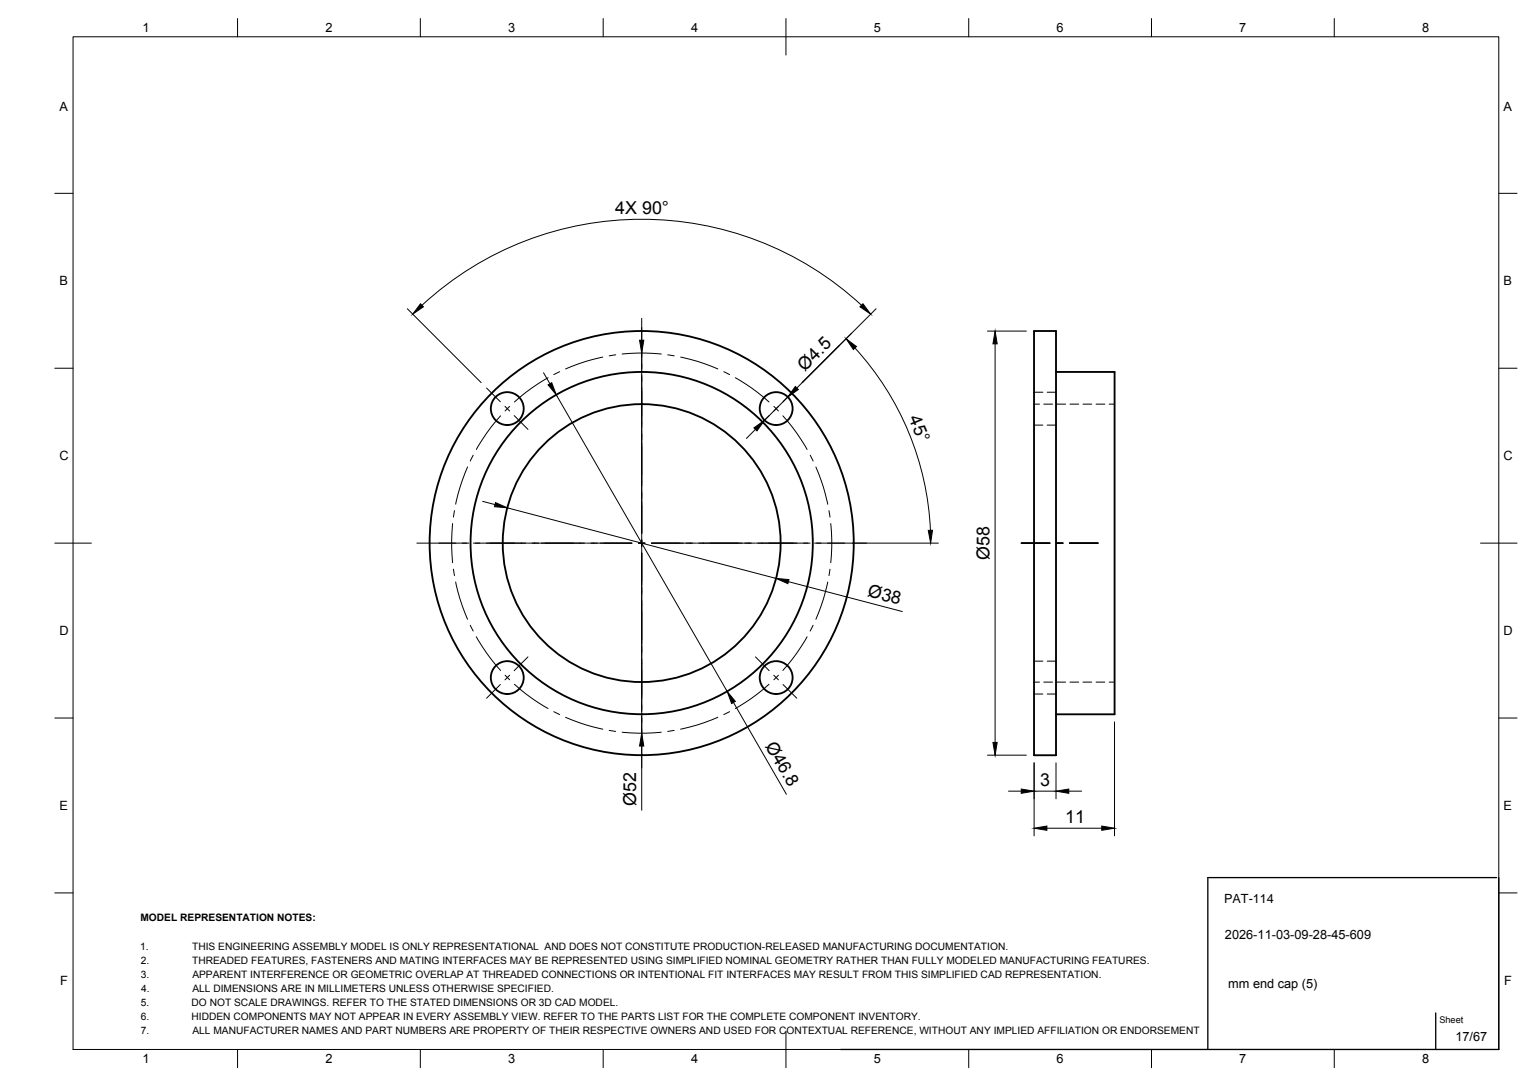
ISO-10303-21;
HEADER;
/* Generated by software containing ST-Developer
 * from STEP Tools, Inc. (www.steptools.com) 
 */

FILE_DESCRIPTION(
/* description */ ('Two-stage gear reducer in split housing'),
/* implementation_level */ '2;1');

FILE_NAME(
/* name */ 'mm end cap (5).step',
/* time_stamp */ '2026-10-28T03:22:31-07:00',
/* author */ (''),
/* organization */ (''),
/* preprocessor_version */ 'ST-DEVELOPER v20.2',
/* originating_system */ 'Autodesk Translation Framework v15.17.0.0',
/* authorisation */ '');

FILE_SCHEMA (('AUTOMOTIVE_DESIGN { 1 0 10303 214 3 1 1 }'));
ENDSEC;

DATA;
#10=MECHANICAL_DESIGN_GEOMETRIC_PRESENTATION_REPRESENTATION('',(#1246),#73366);
#1134=SHAPE_REPRESENTATION_RELATIONSHIP('SRR','None',#73621,#1190);
#1190=ADVANCED_BREP_SHAPE_REPRESENTATION('',(#1317),#73317);
#1246=STYLED_ITEM('',(#74002),#1317);
#1317=MANIFOLD_SOLID_BREP('Body1',#16134);
#1499=FACE_BOUND('',#3296,.T.);
#1500=FACE_BOUND('',#3300,.T.);
#1501=FACE_BOUND('',#3301,.T.);
#1502=FACE_BOUND('',#3302,.T.);
#1503=FACE_BOUND('',#3303,.T.);
#1504=FACE_BOUND('',#3304,.T.);
#1505=FACE_BOUND('',#3306,.T.);
#1506=FACE_BOUND('',#3307,.T.);
#1507=FACE_BOUND('',#3308,.T.);
#1508=FACE_BOUND('',#3309,.T.);
#1509=FACE_BOUND('',#3310,.T.);
#1723=PLANE('',#17350);
#1724=PLANE('',#17357);
#1725=PLANE('',#17358);
#2252=FACE_OUTER_BOUND('',#3290,.T.);
#2253=FACE_OUTER_BOUND('',#3291,.T.);
#2254=FACE_OUTER_BOUND('',#3292,.T.);
#2255=FACE_OUTER_BOUND('',#3293,.T.);
#2256=FACE_OUTER_BOUND('',#3294,.T.);
#2257=FACE_OUTER_BOUND('',#3295,.T.);
#2258=FACE_OUTER_BOUND('',#3297,.T.);
#2259=FACE_OUTER_BOUND('',#3298,.T.);
#2260=FACE_OUTER_BOUND('',#3299,.T.);
#2261=FACE_OUTER_BOUND('',#3305,.T.);
#3290=EDGE_LOOP('',(#11617,#11618,#11619,#11620));
#3291=EDGE_LOOP('',(#11621,#11622,#11623,#11624));
#3292=EDGE_LOOP('',(#11625,#11626,#11627,#11628));
#3293=EDGE_LOOP('',(#11629,#11630,#11631,#11632));
#3294=EDGE_LOOP('',(#11633,#11634,#11635,#11636));
#3295=EDGE_LOOP('',(#11637));
#3296=EDGE_LOOP('',(#11638));
#3297=EDGE_LOOP('',(#11639,#11640,#11641,#11642));
#3298=EDGE_LOOP('',(#11643,#11644,#11645,#11646));
#3299=EDGE_LOOP('',(#11647));
#3300=EDGE_LOOP('',(#11648));
#3301=EDGE_LOOP('',(#11649));
#3302=EDGE_LOOP('',(#11650));
#3303=EDGE_LOOP('',(#11651));
#3304=EDGE_LOOP('',(#11652));
#3305=EDGE_LOOP('',(#11653));
#3306=EDGE_LOOP('',(#11654));
#3307=EDGE_LOOP('',(#11655));
#3308=EDGE_LOOP('',(#11656));
#3309=EDGE_LOOP('',(#11657));
#3310=EDGE_LOOP('',(#11658));
#4353=LINE('',#23968,#5377);
#4354=LINE('',#23974,#5378);
#4355=LINE('',#23980,#5379);
#4356=LINE('',#23986,#5380);
#4357=LINE('',#23992,#5381);
#4358=LINE('',#24000,#5382);
#4359=LINE('',#24005,#5383);
#5377=VECTOR('',#19805,0.225);
#5378=VECTOR('',#19812,0.225);
#5379=VECTOR('',#19819,0.225);
#5380=VECTOR('',#19826,0.225);
#5381=VECTOR('',#19833,2.34);
#5382=VECTOR('',#19844,1.9);
#5383=VECTOR('',#19849,2.9);
#6362=CIRCLE('',#17336,0.225);
#6363=CIRCLE('',#17337,0.225);
#6364=CIRCLE('',#17339,0.225);
#6365=CIRCLE('',#17340,0.225);
#6366=CIRCLE('',#17342,0.225);
#6367=CIRCLE('',#17343,0.225);
#6368=CIRCLE('',#17345,0.225);
#6369=CIRCLE('',#17346,0.225);
#6370=CIRCLE('',#17348,2.34);
#6371=CIRCLE('',#17349,2.34);
#6372=CIRCLE('',#17351,1.9);
#6373=CIRCLE('',#17353,1.9);
#6374=CIRCLE('',#17355,2.9);
#6375=CIRCLE('',#17356,2.9);
#7194=VERTEX_POINT('',#23965);
#7195=VERTEX_POINT('',#23967);
#7196=VERTEX_POINT('',#23971);
#7197=VERTEX_POINT('',#23973);
#7198=VERTEX_POINT('',#23977);
#7199=VERTEX_POINT('',#23979);
#7200=VERTEX_POINT('',#23983);
#7201=VERTEX_POINT('',#23985);
#7202=VERTEX_POINT('',#23989);
#7203=VERTEX_POINT('',#23991);
#7204=VERTEX_POINT('',#23995);
#7205=VERTEX_POINT('',#23998);
#7206=VERTEX_POINT('',#24002);
#7207=VERTEX_POINT('',#24004);
#8862=EDGE_CURVE('',#7194,#7194,#6362,.T.);
#8863=EDGE_CURVE('',#7194,#7195,#4353,.T.);
#8864=EDGE_CURVE('',#7195,#7195,#6363,.T.);
#8865=EDGE_CURVE('',#7196,#7196,#6364,.T.);
#8866=EDGE_CURVE('',#7196,#7197,#4354,.T.);
#8867=EDGE_CURVE('',#7197,#7197,#6365,.T.);
#8868=EDGE_CURVE('',#7198,#7198,#6366,.T.);
#8869=EDGE_CURVE('',#7198,#7199,#4355,.T.);
#8870=EDGE_CURVE('',#7199,#7199,#6367,.T.);
#8871=EDGE_CURVE('',#7200,#7200,#6368,.T.);
#8872=EDGE_CURVE('',#7200,#7201,#4356,.T.);
#8873=EDGE_CURVE('',#7201,#7201,#6369,.T.);
#8874=EDGE_CURVE('',#7202,#7202,#6370,.T.);
#8875=EDGE_CURVE('',#7202,#7203,#4357,.T.);
#8876=EDGE_CURVE('',#7203,#7203,#6371,.T.);
#8877=EDGE_CURVE('',#7204,#7204,#6372,.T.);
#8878=EDGE_CURVE('',#7205,#7205,#6373,.T.);
#8879=EDGE_CURVE('',#7205,#7204,#4358,.T.);
#8880=EDGE_CURVE('',#7206,#7206,#6374,.T.);
#8881=EDGE_CURVE('',#7206,#7207,#4359,.T.);
#8882=EDGE_CURVE('',#7207,#7207,#6375,.T.);
#11617=ORIENTED_EDGE('',*,*,#8862,.F.);
#11618=ORIENTED_EDGE('',*,*,#8863,.T.);
#11619=ORIENTED_EDGE('',*,*,#8864,.F.);
#11620=ORIENTED_EDGE('',*,*,#8863,.F.);
#11621=ORIENTED_EDGE('',*,*,#8865,.F.);
#11622=ORIENTED_EDGE('',*,*,#8866,.T.);
#11623=ORIENTED_EDGE('',*,*,#8867,.F.);
#11624=ORIENTED_EDGE('',*,*,#8866,.F.);
#11625=ORIENTED_EDGE('',*,*,#8868,.F.);
#11626=ORIENTED_EDGE('',*,*,#8869,.T.);
#11627=ORIENTED_EDGE('',*,*,#8870,.F.);
#11628=ORIENTED_EDGE('',*,*,#8869,.F.);
#11629=ORIENTED_EDGE('',*,*,#8871,.F.);
#11630=ORIENTED_EDGE('',*,*,#8872,.T.);
#11631=ORIENTED_EDGE('',*,*,#8873,.F.);
#11632=ORIENTED_EDGE('',*,*,#8872,.F.);
#11633=ORIENTED_EDGE('',*,*,#8874,.F.);
#11634=ORIENTED_EDGE('',*,*,#8875,.T.);
#11635=ORIENTED_EDGE('',*,*,#8876,.T.);
#11636=ORIENTED_EDGE('',*,*,#8875,.F.);
#11637=ORIENTED_EDGE('',*,*,#8876,.F.);
#11638=ORIENTED_EDGE('',*,*,#8877,.F.);
#11639=ORIENTED_EDGE('',*,*,#8878,.F.);
#11640=ORIENTED_EDGE('',*,*,#8879,.T.);
#11641=ORIENTED_EDGE('',*,*,#8877,.T.);
#11642=ORIENTED_EDGE('',*,*,#8879,.F.);
#11643=ORIENTED_EDGE('',*,*,#8880,.F.);
#11644=ORIENTED_EDGE('',*,*,#8881,.T.);
#11645=ORIENTED_EDGE('',*,*,#8882,.T.);
#11646=ORIENTED_EDGE('',*,*,#8881,.F.);
#11647=ORIENTED_EDGE('',*,*,#8880,.T.);
#11648=ORIENTED_EDGE('',*,*,#8878,.T.);
#11649=ORIENTED_EDGE('',*,*,#8873,.T.);
#11650=ORIENTED_EDGE('',*,*,#8870,.T.);
#11651=ORIENTED_EDGE('',*,*,#8867,.T.);
#11652=ORIENTED_EDGE('',*,*,#8864,.T.);
#11653=ORIENTED_EDGE('',*,*,#8882,.F.);
#11654=ORIENTED_EDGE('',*,*,#8874,.T.);
#11655=ORIENTED_EDGE('',*,*,#8871,.T.);
#11656=ORIENTED_EDGE('',*,*,#8868,.T.);
#11657=ORIENTED_EDGE('',*,*,#8865,.T.);
#11658=ORIENTED_EDGE('',*,*,#8862,.T.);
#15036=CYLINDRICAL_SURFACE('',#17335,0.225);
#15037=CYLINDRICAL_SURFACE('',#17338,0.225);
#15038=CYLINDRICAL_SURFACE('',#17341,0.225);
#15039=CYLINDRICAL_SURFACE('',#17344,0.225);
#15040=CYLINDRICAL_SURFACE('',#17347,2.34);
#15041=CYLINDRICAL_SURFACE('',#17352,1.9);
#15042=CYLINDRICAL_SURFACE('',#17354,2.9);
#15459=ADVANCED_FACE('',(#2252),#15036,.F.);
#15460=ADVANCED_FACE('',(#2253),#15037,.F.);
#15461=ADVANCED_FACE('',(#2254),#15038,.F.);
#15462=ADVANCED_FACE('',(#2255),#15039,.F.);
#15463=ADVANCED_FACE('',(#2256),#15040,.T.);
#15464=ADVANCED_FACE('',(#2257,#1499),#1723,.F.);
#15465=ADVANCED_FACE('',(#2258),#15041,.F.);
#15466=ADVANCED_FACE('',(#2259),#15042,.T.);
#15467=ADVANCED_FACE('',(#2260,#1500,#1501,#1502,#1503,#1504),#1724,.T.);
#15468=ADVANCED_FACE('',(#2261,#1505,#1506,#1507,#1508,#1509),#1725,.F.);
#16134=CLOSED_SHELL('',(#15459,#15460,#15461,#15462,#15463,#15464,#15465,
#15466,#15467,#15468));
#17334=AXIS2_PLACEMENT_3D('',#23963,#19799,#19800);
#17335=AXIS2_PLACEMENT_3D('',#23964,#19801,#19802);
#17336=AXIS2_PLACEMENT_3D('',#23966,#19803,#19804);
#17337=AXIS2_PLACEMENT_3D('',#23969,#19806,#19807);
#17338=AXIS2_PLACEMENT_3D('',#23970,#19808,#19809);
#17339=AXIS2_PLACEMENT_3D('',#23972,#19810,#19811);
#17340=AXIS2_PLACEMENT_3D('',#23975,#19813,#19814);
#17341=AXIS2_PLACEMENT_3D('',#23976,#19815,#19816);
#17342=AXIS2_PLACEMENT_3D('',#23978,#19817,#19818);
#17343=AXIS2_PLACEMENT_3D('',#23981,#19820,#19821);
#17344=AXIS2_PLACEMENT_3D('',#23982,#19822,#19823);
#17345=AXIS2_PLACEMENT_3D('',#23984,#19824,#19825);
#17346=AXIS2_PLACEMENT_3D('',#23987,#19827,#19828);
#17347=AXIS2_PLACEMENT_3D('',#23988,#19829,#19830);
#17348=AXIS2_PLACEMENT_3D('',#23990,#19831,#19832);
#17349=AXIS2_PLACEMENT_3D('',#23993,#19834,#19835);
#17350=AXIS2_PLACEMENT_3D('',#23994,#19836,#19837);
#17351=AXIS2_PLACEMENT_3D('',#23996,#19838,#19839);
#17352=AXIS2_PLACEMENT_3D('',#23997,#19840,#19841);
#17353=AXIS2_PLACEMENT_3D('',#23999,#19842,#19843);
#17354=AXIS2_PLACEMENT_3D('',#24001,#19845,#19846);
#17355=AXIS2_PLACEMENT_3D('',#24003,#19847,#19848);
#17356=AXIS2_PLACEMENT_3D('',#24006,#19850,#19851);
#17357=AXIS2_PLACEMENT_3D('',#24007,#19852,#19853);
#17358=AXIS2_PLACEMENT_3D('',#24008,#19854,#19855);
#19799=DIRECTION('axis',(0.,0.,1.));
#19800=DIRECTION('refdir',(1.,0.,0.));
#19801=DIRECTION('center_axis',(0.,1.,0.));
#19802=DIRECTION('ref_axis',(1.,0.,0.));
#19803=DIRECTION('center_axis',(0.,1.,0.));
#19804=DIRECTION('ref_axis',(1.,0.,0.));
#19805=DIRECTION('',(0.,1.,0.));
#19806=DIRECTION('center_axis',(0.,-1.,0.));
#19807=DIRECTION('ref_axis',(1.,0.,0.));
#19808=DIRECTION('center_axis',(0.,1.,0.));
#19809=DIRECTION('ref_axis',(1.,0.,0.));
#19810=DIRECTION('center_axis',(0.,1.,0.));
#19811=DIRECTION('ref_axis',(1.,0.,0.));
#19812=DIRECTION('',(0.,1.,0.));
#19813=DIRECTION('center_axis',(0.,-1.,0.));
#19814=DIRECTION('ref_axis',(1.,0.,0.));
#19815=DIRECTION('center_axis',(0.,1.,0.));
#19816=DIRECTION('ref_axis',(1.,0.,0.));
#19817=DIRECTION('center_axis',(0.,1.,0.));
#19818=DIRECTION('ref_axis',(1.,0.,0.));
#19819=DIRECTION('',(0.,1.,0.));
#19820=DIRECTION('center_axis',(0.,-1.,0.));
#19821=DIRECTION('ref_axis',(1.,0.,0.));
#19822=DIRECTION('center_axis',(0.,1.,0.));
#19823=DIRECTION('ref_axis',(1.,0.,0.));
#19824=DIRECTION('center_axis',(0.,1.,0.));
#19825=DIRECTION('ref_axis',(1.,0.,0.));
#19826=DIRECTION('',(0.,1.,0.));
#19827=DIRECTION('center_axis',(0.,-1.,0.));
#19828=DIRECTION('ref_axis',(1.,0.,0.));
#19829=DIRECTION('center_axis',(0.,1.,0.));
#19830=DIRECTION('ref_axis',(1.,0.,0.));
#19831=DIRECTION('center_axis',(0.,1.,0.));
#19832=DIRECTION('ref_axis',(1.,0.,0.));
#19833=DIRECTION('',(0.,-1.,0.));
#19834=DIRECTION('center_axis',(0.,1.,0.));
#19835=DIRECTION('ref_axis',(1.,0.,0.));
#19836=DIRECTION('center_axis',(0.,1.,0.));
#19837=DIRECTION('ref_axis',(1.,0.,0.));
#19838=DIRECTION('center_axis',(0.,-1.,0.));
#19839=DIRECTION('ref_axis',(1.,0.,0.));
#19840=DIRECTION('center_axis',(0.,1.,0.));
#19841=DIRECTION('ref_axis',(1.,0.,0.));
#19842=DIRECTION('center_axis',(0.,-1.,0.));
#19843=DIRECTION('ref_axis',(1.,0.,0.));
#19844=DIRECTION('',(0.,-1.,0.));
#19845=DIRECTION('center_axis',(0.,1.,0.));
#19846=DIRECTION('ref_axis',(1.,0.,0.));
#19847=DIRECTION('center_axis',(0.,1.,0.));
#19848=DIRECTION('ref_axis',(1.,0.,0.));
#19849=DIRECTION('',(0.,-1.,0.));
#19850=DIRECTION('center_axis',(0.,1.,0.));
#19851=DIRECTION('ref_axis',(1.,0.,0.));
#19852=DIRECTION('center_axis',(0.,1.,0.));
#19853=DIRECTION('ref_axis',(1.,0.,0.));
#19854=DIRECTION('center_axis',(0.,1.,0.));
#19855=DIRECTION('ref_axis',(1.,0.,0.));
#23963=CARTESIAN_POINT('',(0.,0.,0.));
#23964=CARTESIAN_POINT('Origin',(10.161522368915,7.4,8.16152236891498));
#23965=CARTESIAN_POINT('',(9.93652236891498,7.5,8.16152236891498));
#23966=CARTESIAN_POINT('Origin',(10.161522368915,7.5,8.16152236891498));
#23967=CARTESIAN_POINT('',(9.93652236891498,7.8,8.16152236891498));
#23968=CARTESIAN_POINT('',(9.93652236891498,7.4,8.16152236891498));
#23969=CARTESIAN_POINT('Origin',(10.161522368915,7.8,8.16152236891498));
#23970=CARTESIAN_POINT('Origin',(10.161522368915,7.4,11.838477631085));
#23971=CARTESIAN_POINT('',(9.93652236891498,7.5,11.838477631085));
#23972=CARTESIAN_POINT('Origin',(10.161522368915,7.5,11.838477631085));
#23973=CARTESIAN_POINT('',(9.93652236891498,7.8,11.838477631085));
#23974=CARTESIAN_POINT('',(9.93652236891498,7.4,11.838477631085));
#23975=CARTESIAN_POINT('Origin',(10.161522368915,7.8,11.838477631085));
#23976=CARTESIAN_POINT('Origin',(13.838477631085,7.4,11.838477631085));
#23977=CARTESIAN_POINT('',(13.613477631085,7.5,11.838477631085));
#23978=CARTESIAN_POINT('Origin',(13.838477631085,7.5,11.838477631085));
#23979=CARTESIAN_POINT('',(13.613477631085,7.8,11.838477631085));
#23980=CARTESIAN_POINT('',(13.613477631085,7.4,11.838477631085));
#23981=CARTESIAN_POINT('Origin',(13.838477631085,7.8,11.838477631085));
#23982=CARTESIAN_POINT('Origin',(13.838477631085,7.4,8.16152236891498));
#23983=CARTESIAN_POINT('',(13.613477631085,7.5,8.16152236891498));
#23984=CARTESIAN_POINT('Origin',(13.838477631085,7.5,8.16152236891498));
#23985=CARTESIAN_POINT('',(13.613477631085,7.8,8.16152236891498));
#23986=CARTESIAN_POINT('',(13.613477631085,7.4,8.16152236891498));
#23987=CARTESIAN_POINT('Origin',(13.838477631085,7.8,8.16152236891498));
#23988=CARTESIAN_POINT('Origin',(12.,6.7,10.));
#23989=CARTESIAN_POINT('',(9.66,7.5,10.));
#23990=CARTESIAN_POINT('Origin',(12.,7.5,10.));
#23991=CARTESIAN_POINT('',(9.66,6.7,10.));
#23992=CARTESIAN_POINT('',(9.66,6.7,10.));
#23993=CARTESIAN_POINT('Origin',(12.,6.7,10.));
#23994=CARTESIAN_POINT('Origin',(12.,6.7,10.));
#23995=CARTESIAN_POINT('',(10.1,6.7,10.));
#23996=CARTESIAN_POINT('Origin',(12.,6.7,10.));
#23997=CARTESIAN_POINT('Origin',(12.,7.5,10.));
#23998=CARTESIAN_POINT('',(10.1,7.8,10.));
#23999=CARTESIAN_POINT('Origin',(12.,7.8,10.));
#24000=CARTESIAN_POINT('',(10.1,7.5,10.));
#24001=CARTESIAN_POINT('Origin',(12.,7.5,10.));
#24002=CARTESIAN_POINT('',(9.1,7.8,10.));
#24003=CARTESIAN_POINT('Origin',(12.,7.8,10.));
#24004=CARTESIAN_POINT('',(9.1,7.5,10.));
#24005=CARTESIAN_POINT('',(9.1,7.5,10.));
#24006=CARTESIAN_POINT('Origin',(12.,7.5,10.));
#24007=CARTESIAN_POINT('Origin',(12.,7.8,10.));
#24008=CARTESIAN_POINT('Origin',(12.,7.5,10.));
#73253=UNCERTAINTY_MEASURE_WITH_UNIT(LENGTH_MEASURE(0.001),#73367,
'DISTANCE_ACCURACY_VALUE',
'Maximum model space distance between geometric entities at asserted c
onnectivities');
#73302=UNCERTAINTY_MEASURE_WITH_UNIT(LENGTH_MEASURE(0.001),#73367,
'DISTANCE_ACCURACY_VALUE',
'Maximum model space distance between geometric entities at asserted c
onnectivities');
#73317=(
GEOMETRIC_REPRESENTATION_CONTEXT(3)
GLOBAL_UNCERTAINTY_ASSIGNED_CONTEXT((#73253))
GLOBAL_UNIT_ASSIGNED_CONTEXT((#73367,#73369,#73370))
REPRESENTATION_CONTEXT('','3D')
);
#73366=(
GEOMETRIC_REPRESENTATION_CONTEXT(3)
GLOBAL_UNCERTAINTY_ASSIGNED_CONTEXT((#73302))
GLOBAL_UNIT_ASSIGNED_CONTEXT((#73367,#73369,#73370))
REPRESENTATION_CONTEXT('','3D')
);
#73367=(
LENGTH_UNIT()
NAMED_UNIT(*)
SI_UNIT(.CENTI.,.METRE.)
);
#73369=(
NAMED_UNIT(*)
PLANE_ANGLE_UNIT()
SI_UNIT($,.RADIAN.)
);
#73370=(
NAMED_UNIT(*)
SI_UNIT($,.STERADIAN.)
SOLID_ANGLE_UNIT()
);
#73385=SHAPE_DEFINITION_REPRESENTATION(#73448,#73621);
#73448=PRODUCT_DEFINITION_SHAPE('',$,#73685);
#73621=SHAPE_REPRESENTATION('',(#17334),#73317);
#73670=PRODUCT_DEFINITION_CONTEXT('part definition',#73861,'design');
#73685=PRODUCT_DEFINITION('mm end cap (5)','mm end cap (5)',#73748,#73670);
#73748=PRODUCT_DEFINITION_FORMATION('',$,#73877);
#73861=APPLICATION_CONTEXT(
'Core Data for Automotive Mechanical Design Process');
#73862=PRODUCT_CONTEXT('part definition',#73861,'mechanical');
#73877=PRODUCT('mm end cap (5)','mm end cap (5)','mm end cap (5)',(#73862));
#73996=COLOUR_RGB('Off White',0.89,0.88,0.83);
#73997=FILL_AREA_STYLE_COLOUR('',#73996);
#73998=FILL_AREA_STYLE('',(#73997));
#73999=SURFACE_STYLE_FILL_AREA(#73998);
#74000=SURFACE_SIDE_STYLE('',(#73999));
#74001=SURFACE_STYLE_USAGE(.BOTH.,#74000);
#74002=PRESENTATION_STYLE_ASSIGNMENT((#74001));
ENDSEC;
END-ISO-10303-21;
